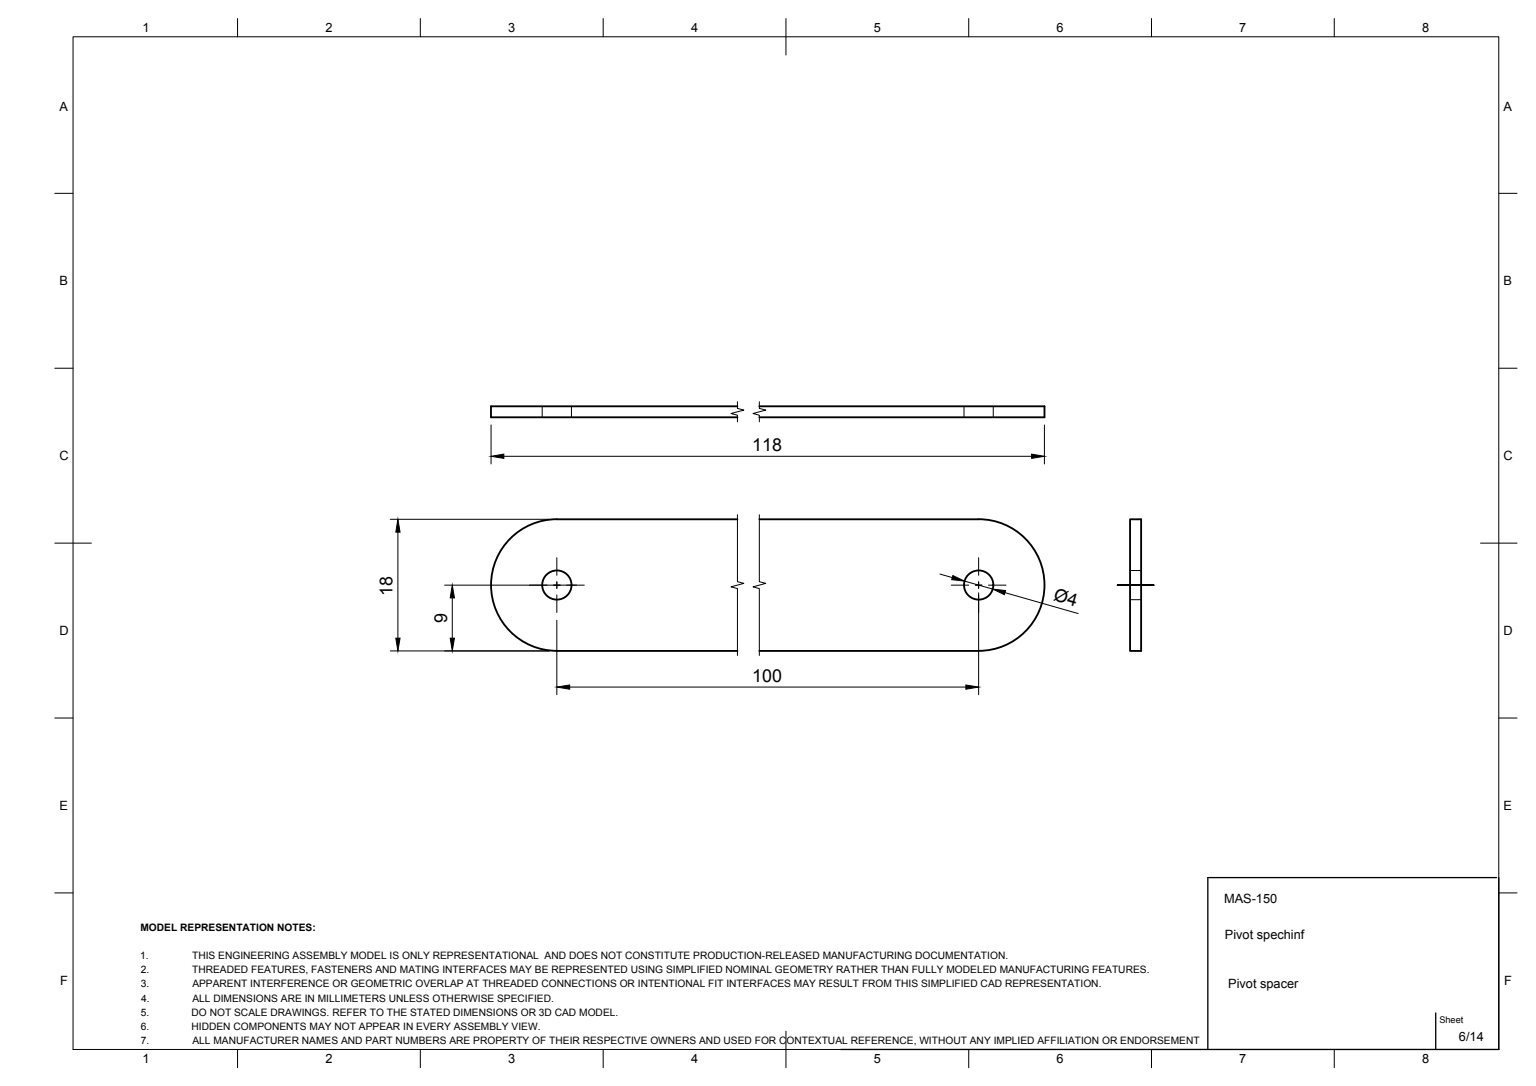
ISO-10303-21;
HEADER;
/* Generated by software containing ST-Developer
 * from STEP Tools, Inc. (www.steptools.com) 
 */

FILE_DESCRIPTION(
/* description */ ('STEP AP203'),
/* implementation_level */ '2;1');

FILE_NAME(
/* name */ 'Pivot spacer.step',
/* time_stamp */ '2026-11-08T21:40:52-08:00',
/* author */ (''),
/* organization */ (''),
/* preprocessor_version */ 'ST-DEVELOPER v20.2',
/* originating_system */ 'Autodesk Translation Framework v15.17.0.0',
/* authorisation */ '');

FILE_SCHEMA (('AUTOMOTIVE_DESIGN { 1 0 10303 214 3 1 1 }'));
ENDSEC;

DATA;
#10=MECHANICAL_DESIGN_GEOMETRIC_PRESENTATION_REPRESENTATION('',(#193),#12137);
#171=SHAPE_REPRESENTATION_RELATIONSHIP('SRR','None',#12195,#182);
#182=ADVANCED_BREP_SHAPE_REPRESENTATION('',(#204),#12136);
#193=STYLED_ITEM('',(#12253),#204);
#204=MANIFOLD_SOLID_BREP('Body1',#1838);
#228=FACE_BOUND('',#728,.T.);
#229=FACE_BOUND('',#729,.T.);
#230=FACE_BOUND('',#731,.T.);
#231=FACE_BOUND('',#732,.T.);
#272=PLANE('',#2138);
#273=PLANE('',#2141);
#274=PLANE('',#2145);
#275=PLANE('',#2147);
#360=LINE('',#12064,#454);
#361=LINE('',#12070,#455);
#362=LINE('',#12077,#456);
#363=LINE('',#12080,#457);
#364=LINE('',#12086,#458);
#365=LINE('',#12089,#459);
#366=LINE('',#12091,#460);
#367=LINE('',#12092,#461);
#368=LINE('',#12094,#462);
#369=LINE('',#12096,#463);
#454=VECTOR('',#2590,2.);
#455=VECTOR('',#2597,2.00000000000001);
#456=VECTOR('',#2604,1000.);
#457=VECTOR('',#2607,1000.);
#458=VECTOR('',#2612,1000.);
#459=VECTOR('',#2615,1000.);
#460=VECTOR('',#2618,1000.);
#461=VECTOR('',#2619,1000.);
#462=VECTOR('',#2622,1000.);
#463=VECTOR('',#2625,1000.);
#486=CYLINDRICAL_SURFACE('',#2132,2.);
#487=CYLINDRICAL_SURFACE('',#2135,2.00000000000001);
#488=CYLINDRICAL_SURFACE('',#2144,9.00000000000003);
#489=CYLINDRICAL_SURFACE('',#2146,9.00000000000005);
#592=FACE_OUTER_BOUND('',#725,.T.);
#593=FACE_OUTER_BOUND('',#726,.T.);
#594=FACE_OUTER_BOUND('',#727,.T.);
#595=FACE_OUTER_BOUND('',#730,.T.);
#596=FACE_OUTER_BOUND('',#733,.T.);
#597=FACE_OUTER_BOUND('',#734,.T.);
#598=FACE_OUTER_BOUND('',#735,.T.);
#599=FACE_OUTER_BOUND('',#736,.T.);
#725=EDGE_LOOP('',(#1671,#1672,#1673,#1674));
#726=EDGE_LOOP('',(#1675,#1676,#1677,#1678));
#727=EDGE_LOOP('',(#1679,#1680,#1681,#1682));
#728=EDGE_LOOP('',(#1683));
#729=EDGE_LOOP('',(#1684));
#730=EDGE_LOOP('',(#1685,#1686,#1687,#1688));
#731=EDGE_LOOP('',(#1689));
#732=EDGE_LOOP('',(#1690));
#733=EDGE_LOOP('',(#1691,#1692,#1693,#1694));
#734=EDGE_LOOP('',(#1695,#1696,#1697,#1698));
#735=EDGE_LOOP('',(#1699,#1700,#1701,#1702));
#736=EDGE_LOOP('',(#1703,#1704,#1705,#1706));
#816=CIRCLE('',#2133,2.);
#817=CIRCLE('',#2134,2.);
#818=CIRCLE('',#2136,2.00000000000001);
#819=CIRCLE('',#2137,2.00000000000001);
#820=CIRCLE('',#2139,9.00000000000003);
#821=CIRCLE('',#2140,9.00000000000005);
#822=CIRCLE('',#2142,9.00000000000003);
#823=CIRCLE('',#2143,9.00000000000005);
#969=VERTEX_POINT('',#12061);
#970=VERTEX_POINT('',#12063);
#971=VERTEX_POINT('',#12067);
#972=VERTEX_POINT('',#12069);
#973=VERTEX_POINT('',#12073);
#974=VERTEX_POINT('',#12074);
#975=VERTEX_POINT('',#12076);
#976=VERTEX_POINT('',#12078);
#977=VERTEX_POINT('',#12082);
#978=VERTEX_POINT('',#12083);
#979=VERTEX_POINT('',#12085);
#980=VERTEX_POINT('',#12087);
#1205=EDGE_CURVE('',#969,#969,#816,.T.);
#1206=EDGE_CURVE('',#969,#970,#360,.T.);
#1207=EDGE_CURVE('',#970,#970,#817,.T.);
#1208=EDGE_CURVE('',#971,#971,#818,.T.);
#1209=EDGE_CURVE('',#971,#972,#361,.T.);
#1210=EDGE_CURVE('',#972,#972,#819,.T.);
#1211=EDGE_CURVE('',#973,#974,#820,.T.);
#1212=EDGE_CURVE('',#974,#975,#362,.T.);
#1213=EDGE_CURVE('',#975,#976,#821,.T.);
#1214=EDGE_CURVE('',#976,#973,#363,.T.);
#1215=EDGE_CURVE('',#977,#978,#822,.T.);
#1216=EDGE_CURVE('',#979,#977,#364,.T.);
#1217=EDGE_CURVE('',#980,#979,#823,.T.);
#1218=EDGE_CURVE('',#978,#980,#365,.T.);
#1219=EDGE_CURVE('',#974,#978,#366,.T.);
#1220=EDGE_CURVE('',#973,#977,#367,.T.);
#1221=EDGE_CURVE('',#975,#980,#368,.T.);
#1222=EDGE_CURVE('',#976,#979,#369,.T.);
#1671=ORIENTED_EDGE('',*,*,#1205,.T.);
#1672=ORIENTED_EDGE('',*,*,#1206,.T.);
#1673=ORIENTED_EDGE('',*,*,#1207,.F.);
#1674=ORIENTED_EDGE('',*,*,#1206,.F.);
#1675=ORIENTED_EDGE('',*,*,#1208,.T.);
#1676=ORIENTED_EDGE('',*,*,#1209,.T.);
#1677=ORIENTED_EDGE('',*,*,#1210,.F.);
#1678=ORIENTED_EDGE('',*,*,#1209,.F.);
#1679=ORIENTED_EDGE('',*,*,#1211,.T.);
#1680=ORIENTED_EDGE('',*,*,#1212,.T.);
#1681=ORIENTED_EDGE('',*,*,#1213,.T.);
#1682=ORIENTED_EDGE('',*,*,#1214,.T.);
#1683=ORIENTED_EDGE('',*,*,#1205,.F.);
#1684=ORIENTED_EDGE('',*,*,#1208,.F.);
#1685=ORIENTED_EDGE('',*,*,#1215,.F.);
#1686=ORIENTED_EDGE('',*,*,#1216,.F.);
#1687=ORIENTED_EDGE('',*,*,#1217,.F.);
#1688=ORIENTED_EDGE('',*,*,#1218,.F.);
#1689=ORIENTED_EDGE('',*,*,#1210,.T.);
#1690=ORIENTED_EDGE('',*,*,#1207,.T.);
#1691=ORIENTED_EDGE('',*,*,#1215,.T.);
#1692=ORIENTED_EDGE('',*,*,#1219,.F.);
#1693=ORIENTED_EDGE('',*,*,#1211,.F.);
#1694=ORIENTED_EDGE('',*,*,#1220,.T.);
#1695=ORIENTED_EDGE('',*,*,#1218,.T.);
#1696=ORIENTED_EDGE('',*,*,#1221,.F.);
#1697=ORIENTED_EDGE('',*,*,#1212,.F.);
#1698=ORIENTED_EDGE('',*,*,#1219,.T.);
#1699=ORIENTED_EDGE('',*,*,#1217,.T.);
#1700=ORIENTED_EDGE('',*,*,#1222,.F.);
#1701=ORIENTED_EDGE('',*,*,#1213,.F.);
#1702=ORIENTED_EDGE('',*,*,#1221,.T.);
#1703=ORIENTED_EDGE('',*,*,#1216,.T.);
#1704=ORIENTED_EDGE('',*,*,#1220,.F.);
#1705=ORIENTED_EDGE('',*,*,#1214,.F.);
#1706=ORIENTED_EDGE('',*,*,#1222,.T.);
#1820=ADVANCED_FACE('',(#592),#486,.F.);
#1821=ADVANCED_FACE('',(#593),#487,.F.);
#1822=ADVANCED_FACE('',(#594,#228,#229),#272,.T.);
#1823=ADVANCED_FACE('',(#595,#230,#231),#273,.F.);
#1824=ADVANCED_FACE('',(#596),#488,.T.);
#1825=ADVANCED_FACE('',(#597),#274,.F.);
#1826=ADVANCED_FACE('',(#598),#489,.T.);
#1827=ADVANCED_FACE('',(#599),#275,.F.);
#1838=CLOSED_SHELL('',(#1820,#1821,#1822,#1823,#1824,#1825,#1826,#1827));
#2131=AXIS2_PLACEMENT_3D('',#12059,#2584,#2585);
#2132=AXIS2_PLACEMENT_3D('',#12060,#2586,#2587);
#2133=AXIS2_PLACEMENT_3D('',#12062,#2588,#2589);
#2134=AXIS2_PLACEMENT_3D('',#12065,#2591,#2592);
#2135=AXIS2_PLACEMENT_3D('',#12066,#2593,#2594);
#2136=AXIS2_PLACEMENT_3D('',#12068,#2595,#2596);
#2137=AXIS2_PLACEMENT_3D('',#12071,#2598,#2599);
#2138=AXIS2_PLACEMENT_3D('',#12072,#2600,#2601);
#2139=AXIS2_PLACEMENT_3D('',#12075,#2602,#2603);
#2140=AXIS2_PLACEMENT_3D('',#12079,#2605,#2606);
#2141=AXIS2_PLACEMENT_3D('',#12081,#2608,#2609);
#2142=AXIS2_PLACEMENT_3D('',#12084,#2610,#2611);
#2143=AXIS2_PLACEMENT_3D('',#12088,#2613,#2614);
#2144=AXIS2_PLACEMENT_3D('',#12090,#2616,#2617);
#2145=AXIS2_PLACEMENT_3D('',#12093,#2620,#2621);
#2146=AXIS2_PLACEMENT_3D('',#12095,#2623,#2624);
#2147=AXIS2_PLACEMENT_3D('',#12097,#2626,#2627);
#2584=DIRECTION('axis',(0.,0.,1.));
#2585=DIRECTION('refdir',(1.,0.,0.));
#2586=DIRECTION('center_axis',(0.,-1.,0.));
#2587=DIRECTION('ref_axis',(0.,0.,-1.));
#2588=DIRECTION('center_axis',(0.,1.,0.));
#2589=DIRECTION('ref_axis',(0.,0.,1.));
#2590=DIRECTION('',(0.,-1.,0.));
#2591=DIRECTION('center_axis',(0.,1.,0.));
#2592=DIRECTION('ref_axis',(0.,0.,1.));
#2593=DIRECTION('center_axis',(0.,-1.,0.));
#2594=DIRECTION('ref_axis',(0.,0.,-1.));
#2595=DIRECTION('center_axis',(0.,1.,0.));
#2596=DIRECTION('ref_axis',(0.,0.,1.));
#2597=DIRECTION('',(0.,-1.,0.));
#2598=DIRECTION('center_axis',(0.,1.,0.));
#2599=DIRECTION('ref_axis',(0.,0.,1.));
#2600=DIRECTION('center_axis',(0.,1.,0.));
#2601=DIRECTION('ref_axis',(0.,0.,1.));
#2602=DIRECTION('center_axis',(0.,1.,0.));
#2603=DIRECTION('ref_axis',(0.,0.,1.));
#2604=DIRECTION('',(-1.,0.,-2.42861286636752E-16));
#2605=DIRECTION('center_axis',(0.,1.,0.));
#2606=DIRECTION('ref_axis',(0.,0.,1.));
#2607=DIRECTION('',(1.,0.,-1.38777878078144E-16));
#2608=DIRECTION('center_axis',(0.,1.,0.));
#2609=DIRECTION('ref_axis',(0.,0.,1.));
#2610=DIRECTION('center_axis',(0.,1.,0.));
#2611=DIRECTION('ref_axis',(0.,0.,1.));
#2612=DIRECTION('',(1.,0.,-1.38777878078144E-16));
#2613=DIRECTION('center_axis',(0.,1.,0.));
#2614=DIRECTION('ref_axis',(0.,0.,1.));
#2615=DIRECTION('',(-1.,0.,-2.42861286636752E-16));
#2616=DIRECTION('center_axis',(0.,-1.,0.));
#2617=DIRECTION('ref_axis',(0.,0.,-1.));
#2618=DIRECTION('',(0.,-1.,0.));
#2619=DIRECTION('',(0.,-1.,0.));
#2620=DIRECTION('center_axis',(-2.42861286636752E-16,0.,1.));
#2621=DIRECTION('ref_axis',(1.,0.,2.42861286636752E-16));
#2622=DIRECTION('',(0.,-1.,0.));
#2623=DIRECTION('center_axis',(0.,-1.,0.));
#2624=DIRECTION('ref_axis',(0.,0.,-1.));
#2625=DIRECTION('',(0.,-1.,0.));
#2626=DIRECTION('center_axis',(-1.38777878078144E-16,0.,-1.));
#2627=DIRECTION('ref_axis',(-1.,0.,1.38777878078144E-16));
#12059=CARTESIAN_POINT('',(0.,0.,0.));
#12060=CARTESIAN_POINT('Origin',(72.6432649512037,1.5,-2.848178441575));
#12061=CARTESIAN_POINT('',(72.6432649512037,1.5,-0.848178441574995));
#12062=CARTESIAN_POINT('Origin',(72.6432649512037,1.5,-2.848178441575));
#12063=CARTESIAN_POINT('',(72.6432649512037,0.,-0.848178441574995));
#12064=CARTESIAN_POINT('',(72.6432649512037,1.5,-0.848178441575));
#12065=CARTESIAN_POINT('Origin',(72.6432649512037,0.,-2.848178441575));
#12066=CARTESIAN_POINT('Origin',(-27.3567350487966,1.5,-2.84817844157499));
#12067=CARTESIAN_POINT('',(-27.3567350487966,1.5,-0.848178441574983));
#12068=CARTESIAN_POINT('Origin',(-27.3567350487966,1.5,-2.84817844157499));
#12069=CARTESIAN_POINT('',(-27.3567350487966,0.,-0.848178441574983));
#12070=CARTESIAN_POINT('',(-27.3567350487966,1.5,-0.84817844157498));
#12071=CARTESIAN_POINT('Origin',(-27.3567350487966,0.,-2.84817844157499));
#12072=CARTESIAN_POINT('Origin',(72.6432649512037,1.5,-2.848178441575));
#12073=CARTESIAN_POINT('',(72.6432649512037,1.5,6.15182155842503));
#12074=CARTESIAN_POINT('',(72.6432649512038,1.5,-11.848178441575));
#12075=CARTESIAN_POINT('Origin',(72.6432649512037,1.5,-2.848178441575));
#12076=CARTESIAN_POINT('',(-27.3567350487966,1.5,-11.8481784415751));
#12077=CARTESIAN_POINT('',(72.6432649512038,1.5,-11.848178441575));
#12078=CARTESIAN_POINT('',(-27.3567350487967,1.5,6.15182155842505));
#12079=CARTESIAN_POINT('Origin',(-27.3567350487966,1.5,-2.84817844157499));
#12080=CARTESIAN_POINT('',(72.6432649512037,1.5,6.15182155842503));
#12081=CARTESIAN_POINT('Origin',(72.6432649512037,0.,-2.848178441575));
#12082=CARTESIAN_POINT('',(72.6432649512037,0.,6.15182155842503));
#12083=CARTESIAN_POINT('',(72.6432649512038,0.,-11.848178441575));
#12084=CARTESIAN_POINT('Origin',(72.6432649512037,0.,-2.848178441575));
#12085=CARTESIAN_POINT('',(-27.3567350487967,0.,6.15182155842505));
#12086=CARTESIAN_POINT('',(72.6432649512037,0.,6.15182155842503));
#12087=CARTESIAN_POINT('',(-27.3567350487966,0.,-11.8481784415751));
#12088=CARTESIAN_POINT('Origin',(-27.3567350487966,0.,-2.84817844157499));
#12089=CARTESIAN_POINT('',(72.6432649512038,0.,-11.848178441575));
#12090=CARTESIAN_POINT('Origin',(72.6432649512037,1.5,-2.848178441575));
#12091=CARTESIAN_POINT('',(72.6432649512038,1.5,-11.848178441575));
#12092=CARTESIAN_POINT('',(72.6432649512037,1.5,6.15182155842503));
#12093=CARTESIAN_POINT('Origin',(72.6432649512038,1.5,-11.848178441575));
#12094=CARTESIAN_POINT('',(-27.3567350487966,1.5,-11.8481784415751));
#12095=CARTESIAN_POINT('Origin',(-27.3567350487966,1.5,-2.84817844157499));
#12096=CARTESIAN_POINT('',(-27.3567350487967,1.5,6.15182155842505));
#12097=CARTESIAN_POINT('Origin',(72.6432649512037,1.5,6.15182155842503));
#12122=UNCERTAINTY_MEASURE_WITH_UNIT(LENGTH_MEASURE(0.01),#12138,
'DISTANCE_ACCURACY_VALUE',
'Maximum model space distance between geometric entities at asserted c
onnectivities');
#12123=UNCERTAINTY_MEASURE_WITH_UNIT(LENGTH_MEASURE(0.01),#12138,
'DISTANCE_ACCURACY_VALUE',
'Maximum model space distance between geometric entities at asserted c
onnectivities');
#12136=(
GEOMETRIC_REPRESENTATION_CONTEXT(3)
GLOBAL_UNCERTAINTY_ASSIGNED_CONTEXT((#12122))
GLOBAL_UNIT_ASSIGNED_CONTEXT((#12138,#12140,#12141))
REPRESENTATION_CONTEXT('','3D')
);
#12137=(
GEOMETRIC_REPRESENTATION_CONTEXT(3)
GLOBAL_UNCERTAINTY_ASSIGNED_CONTEXT((#12123))
GLOBAL_UNIT_ASSIGNED_CONTEXT((#12138,#12140,#12141))
REPRESENTATION_CONTEXT('','3D')
);
#12138=(
LENGTH_UNIT()
NAMED_UNIT(*)
SI_UNIT(.MILLI.,.METRE.)
);
#12140=(
NAMED_UNIT(*)
PLANE_ANGLE_UNIT()
SI_UNIT($,.RADIAN.)
);
#12141=(
NAMED_UNIT(*)
SI_UNIT($,.STERADIAN.)
SOLID_ANGLE_UNIT()
);
#12154=SHAPE_DEFINITION_REPRESENTATION(#12170,#12195);
#12170=PRODUCT_DEFINITION_SHAPE('',$,#12209);
#12195=SHAPE_REPRESENTATION('',(#2131),#12136);
#12196=PRODUCT_DEFINITION_CONTEXT('part definition',#12237,'design');
#12209=PRODUCT_DEFINITION('Pivot spechinf','Pivot spacer',#12222,#12196);
#12222=PRODUCT_DEFINITION_FORMATION('',$,#12251);
#12237=APPLICATION_CONTEXT(
'Core Data for Automotive Mechanical Design Process');
#12238=PRODUCT_CONTEXT('part definition',#12237,'mechanical');
#12251=PRODUCT('Pivot spechinf','Pivot spacer',$,(#12238));
#12253=PRESENTATION_STYLE_ASSIGNMENT((#12255));
#12255=SURFACE_STYLE_USAGE(.BOTH.,#12257);
#12257=SURFACE_SIDE_STYLE('',(#12259));
#12259=SURFACE_STYLE_FILL_AREA(#12261);
#12261=FILL_AREA_STYLE('Opaque(23,69,131)',(#12263));
#12263=FILL_AREA_STYLE_COLOUR('Opaque(23,69,131)',#12265);
#12265=COLOUR_RGB('Opaque(23,69,131)',0.0901960784313725,0.270588235294118,
0.513725490196078);
ENDSEC;
END-ISO-10303-21;
